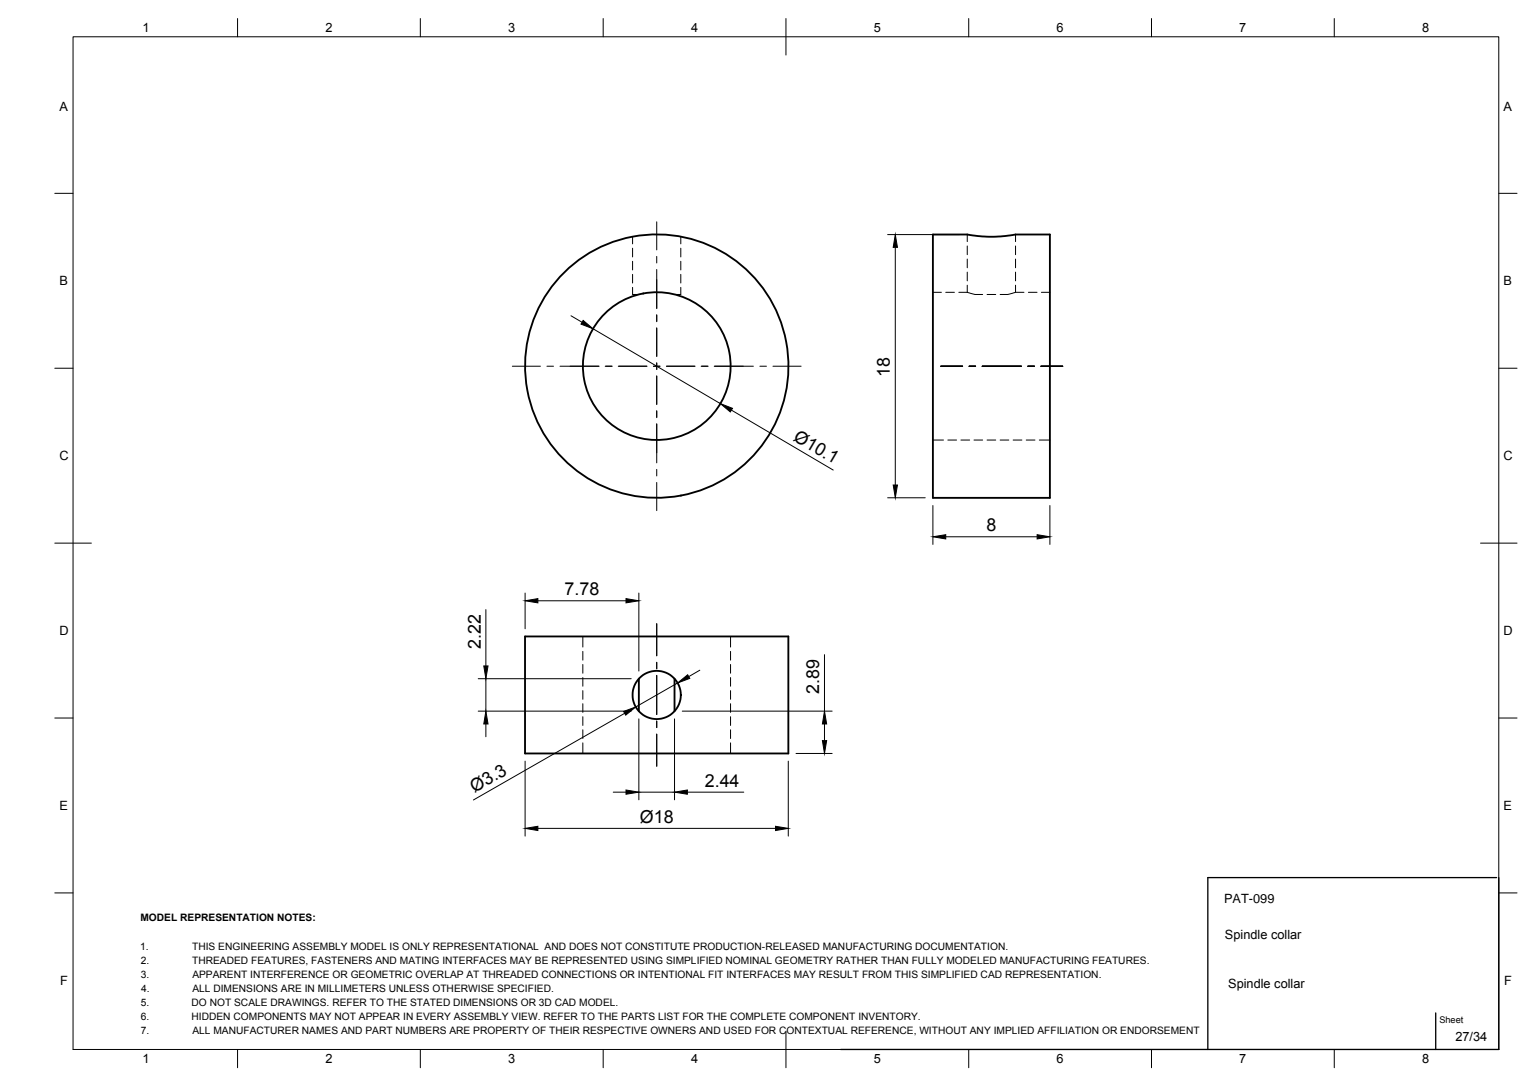
ISO-10303-21;
HEADER;
/* Generated by software containing ST-Developer
 * from STEP Tools, Inc. (www.steptools.com) 
 */

FILE_DESCRIPTION(
/* description */ ('PAT-099'),
/* implementation_level */ '2;1');

FILE_NAME(
/* name */ 'Spindle collar.step',
/* time_stamp */ '2026-10-29T17:25:42-07:00',
/* author */ (''),
/* organization */ (''),
/* preprocessor_version */ 'ST-DEVELOPER v20.2',
/* originating_system */ 'Autodesk Translation Framework v15.17.0.0',
/* authorisation */ '');

FILE_SCHEMA (('AUTOMOTIVE_DESIGN { 1 0 10303 214 3 1 1 }'));
ENDSEC;

DATA;
#10=MECHANICAL_DESIGN_GEOMETRIC_PRESENTATION_REPRESENTATION('',(#349),#11035);
#264=B_SPLINE_CURVE_WITH_KNOTS('',3,(#9974,#9975,#9976,#9977,#9978,#9979,
#9980,#9981,#9982,#9983,#9984,#9985,#9986,#9987),.UNSPECIFIED.,.F.,.F.,
(4,2,2,2,2,2,4),(0.618551524396293,0.626563103102765,0.689203386094988,
0.751843669087211,0.814483952079434,0.877124235071657,0.88513581377813),
 .UNSPECIFIED.);
#265=B_SPLINE_CURVE_WITH_KNOTS('',3,(#9991,#9992,#9993,#9994,#9995,#9996,
#9997,#9998),.UNSPECIFIED.,.F.,.F.,(4,2,2,4),(0.250614556362404,0.313254839354627,
0.37589512234685,0.383906701053323),.UNSPECIFIED.);
#266=B_SPLINE_CURVE_WITH_KNOTS('',3,(#10002,#10003,#10004,#10005,#10006,
#10007,#10008,#10009,#10010,#10011,#10012,#10013,#10014,#10015,#10016,#10017,
#10018,#10019,#10020,#10021,#10022,#10023,#10024,#10025,#10026,#10027),
 .UNSPECIFIED.,.F.,.F.,(4,2,2,2,2,2,2,2,2,2,2,2,4),(0.,0.0623062782223143,
0.124612556444629,0.186916384615149,0.249220212785669,0.31152404095619,
0.37382786912671,0.436134147349024,0.498440425571339,0.560746703793653,
0.623052982015967,0.685356810186488,0.747660638357008),.UNSPECIFIED.);
#267=B_SPLINE_CURVE_WITH_KNOTS('',3,(#10028,#10029,#10030,#10031,#10032,
#10033,#10034,#10035,#10036,#10037),.UNSPECIFIED.,.F.,.F.,(4,2,2,2,4),(0.747660638357008,
0.809964466527528,0.872268294698049,0.934574572920363,0.996880851142677),
 .UNSPECIFIED.);
#268=B_SPLINE_CURVE_WITH_KNOTS('',3,(#10038,#10039,#10040,#10041,#10042,
#10043,#10044,#10045),.UNSPECIFIED.,.F.,.F.,(4,2,2,4),(0.117322411671485,
0.125333990377958,0.187974273370181,0.250614556362404),.UNSPECIFIED.);
#299=SHAPE_REPRESENTATION_RELATIONSHIP('SRR','None',#11169,#324);
#324=ADVANCED_BREP_SHAPE_REPRESENTATION('',(#381),#11019);
#349=STYLED_ITEM('',(#11379),#381);
#381=MANIFOLD_SOLID_BREP('Body1',#4718);
#495=FACE_BOUND('',#1197,.T.);
#496=FACE_BOUND('',#1199,.T.);
#497=FACE_BOUND('',#1201,.T.);
#498=FACE_BOUND('',#1203,.T.);
#597=PLANE('',#5364);
#598=PLANE('',#5368);
#599=PLANE('',#5375);
#600=PLANE('',#5376);
#818=FACE_OUTER_BOUND('',#1193,.T.);
#819=FACE_OUTER_BOUND('',#1194,.T.);
#820=FACE_OUTER_BOUND('',#1195,.T.);
#821=FACE_OUTER_BOUND('',#1196,.T.);
#822=FACE_OUTER_BOUND('',#1198,.T.);
#823=FACE_OUTER_BOUND('',#1200,.T.);
#824=FACE_OUTER_BOUND('',#1202,.T.);
#1193=EDGE_LOOP('',(#3815,#3816));
#1194=EDGE_LOOP('',(#3817,#3818,#3819,#3820,#3821,#3822,#3823,#3824,#3825));
#1195=EDGE_LOOP('',(#3826,#3827));
#1196=EDGE_LOOP('',(#3828,#3829,#3830,#3831));
#1197=EDGE_LOOP('',(#3832,#3833,#3834,#3835,#3836));
#1198=EDGE_LOOP('',(#3837,#3838,#3839,#3840));
#1199=EDGE_LOOP('',(#3841,#3842));
#1200=EDGE_LOOP('',(#3843));
#1201=EDGE_LOOP('',(#3844));
#1202=EDGE_LOOP('',(#3845));
#1203=EDGE_LOOP('',(#3846));
#1491=LINE('',#9970,#1743);
#1492=LINE('',#10000,#1744);
#1493=LINE('',#10047,#1745);
#1494=LINE('',#10052,#1746);
#1495=LINE('',#10058,#1747);
#1743=VECTOR('',#6514,1.);
#1744=VECTOR('',#6521,0.165);
#1745=VECTOR('',#6524,1.);
#1746=VECTOR('',#6529,0.505);
#1747=VECTOR('',#6536,0.9);
#2018=CIRCLE('',#5365,0.165);
#2019=CIRCLE('',#5367,0.165);
#2020=CIRCLE('',#5370,0.505);
#2021=CIRCLE('',#5371,0.505);
#2022=CIRCLE('',#5373,0.9);
#2023=CIRCLE('',#5374,0.9);
#2369=VERTEX_POINT('',#9968);
#2370=VERTEX_POINT('',#9969);
#2371=VERTEX_POINT('',#9973);
#2372=VERTEX_POINT('',#9988);
#2373=VERTEX_POINT('',#9990);
#2374=VERTEX_POINT('',#9999);
#2375=VERTEX_POINT('',#10001);
#2376=VERTEX_POINT('',#10049);
#2377=VERTEX_POINT('',#10051);
#2378=VERTEX_POINT('',#10055);
#2379=VERTEX_POINT('',#10057);
#2884=EDGE_CURVE('',#2369,#2370,#1491,.T.);
#2885=EDGE_CURVE('',#2369,#2370,#2018,.T.);
#2886=EDGE_CURVE('',#2371,#2369,#264,.T.);
#2887=EDGE_CURVE('',#2372,#2371,#2019,.T.);
#2888=EDGE_CURVE('',#2373,#2372,#265,.T.);
#2889=EDGE_CURVE('',#2373,#2374,#1492,.T.);
#2890=EDGE_CURVE('',#2375,#2374,#266,.T.);
#2891=EDGE_CURVE('',#2374,#2375,#267,.T.);
#2892=EDGE_CURVE('',#2370,#2373,#268,.T.);
#2893=EDGE_CURVE('',#2372,#2371,#1493,.T.);
#2894=EDGE_CURVE('',#2376,#2376,#2020,.T.);
#2895=EDGE_CURVE('',#2376,#2377,#1494,.T.);
#2896=EDGE_CURVE('',#2377,#2377,#2021,.T.);
#2897=EDGE_CURVE('',#2378,#2378,#2022,.T.);
#2898=EDGE_CURVE('',#2378,#2379,#1495,.T.);
#2899=EDGE_CURVE('',#2379,#2379,#2023,.T.);
#3815=ORIENTED_EDGE('',*,*,#2884,.F.);
#3816=ORIENTED_EDGE('',*,*,#2885,.T.);
#3817=ORIENTED_EDGE('',*,*,#2886,.F.);
#3818=ORIENTED_EDGE('',*,*,#2887,.F.);
#3819=ORIENTED_EDGE('',*,*,#2888,.F.);
#3820=ORIENTED_EDGE('',*,*,#2889,.T.);
#3821=ORIENTED_EDGE('',*,*,#2890,.F.);
#3822=ORIENTED_EDGE('',*,*,#2891,.F.);
#3823=ORIENTED_EDGE('',*,*,#2889,.F.);
#3824=ORIENTED_EDGE('',*,*,#2892,.F.);
#3825=ORIENTED_EDGE('',*,*,#2885,.F.);
#3826=ORIENTED_EDGE('',*,*,#2893,.F.);
#3827=ORIENTED_EDGE('',*,*,#2887,.T.);
#3828=ORIENTED_EDGE('',*,*,#2894,.F.);
#3829=ORIENTED_EDGE('',*,*,#2895,.T.);
#3830=ORIENTED_EDGE('',*,*,#2896,.T.);
#3831=ORIENTED_EDGE('',*,*,#2895,.F.);
#3832=ORIENTED_EDGE('',*,*,#2892,.T.);
#3833=ORIENTED_EDGE('',*,*,#2888,.T.);
#3834=ORIENTED_EDGE('',*,*,#2893,.T.);
#3835=ORIENTED_EDGE('',*,*,#2886,.T.);
#3836=ORIENTED_EDGE('',*,*,#2884,.T.);
#3837=ORIENTED_EDGE('',*,*,#2897,.F.);
#3838=ORIENTED_EDGE('',*,*,#2898,.T.);
#3839=ORIENTED_EDGE('',*,*,#2899,.T.);
#3840=ORIENTED_EDGE('',*,*,#2898,.F.);
#3841=ORIENTED_EDGE('',*,*,#2890,.T.);
#3842=ORIENTED_EDGE('',*,*,#2891,.T.);
#3843=ORIENTED_EDGE('',*,*,#2897,.T.);
#3844=ORIENTED_EDGE('',*,*,#2894,.T.);
#3845=ORIENTED_EDGE('',*,*,#2899,.F.);
#3846=ORIENTED_EDGE('',*,*,#2896,.F.);
#4390=CYLINDRICAL_SURFACE('',#5366,0.165);
#4391=CYLINDRICAL_SURFACE('',#5369,0.505);
#4392=CYLINDRICAL_SURFACE('',#5372,0.9);
#4583=ADVANCED_FACE('',(#818),#597,.T.);
#4584=ADVANCED_FACE('',(#819),#4390,.F.);
#4585=ADVANCED_FACE('',(#820),#598,.T.);
#4586=ADVANCED_FACE('',(#821,#495),#4391,.F.);
#4587=ADVANCED_FACE('',(#822,#496),#4392,.T.);
#4588=ADVANCED_FACE('',(#823,#497),#599,.T.);
#4589=ADVANCED_FACE('',(#824,#498),#600,.F.);
#4718=CLOSED_SHELL('',(#4583,#4584,#4585,#4586,#4587,#4588,#4589));
#5363=AXIS2_PLACEMENT_3D('',#9966,#6510,#6511);
#5364=AXIS2_PLACEMENT_3D('',#9967,#6512,#6513);
#5365=AXIS2_PLACEMENT_3D('',#9971,#6515,#6516);
#5366=AXIS2_PLACEMENT_3D('',#9972,#6517,#6518);
#5367=AXIS2_PLACEMENT_3D('',#9989,#6519,#6520);
#5368=AXIS2_PLACEMENT_3D('',#10046,#6522,#6523);
#5369=AXIS2_PLACEMENT_3D('',#10048,#6525,#6526);
#5370=AXIS2_PLACEMENT_3D('',#10050,#6527,#6528);
#5371=AXIS2_PLACEMENT_3D('',#10053,#6530,#6531);
#5372=AXIS2_PLACEMENT_3D('',#10054,#6532,#6533);
#5373=AXIS2_PLACEMENT_3D('',#10056,#6534,#6535);
#5374=AXIS2_PLACEMENT_3D('',#10059,#6537,#6538);
#5375=AXIS2_PLACEMENT_3D('',#10060,#6539,#6540);
#5376=AXIS2_PLACEMENT_3D('',#10061,#6541,#6542);
#6510=DIRECTION('axis',(0.,0.,1.));
#6511=DIRECTION('refdir',(1.,0.,0.));
#6512=DIRECTION('center_axis',(1.,0.,0.));
#6513=DIRECTION('ref_axis',(0.,0.,-1.));
#6514=DIRECTION('',(0.,0.,1.));
#6515=DIRECTION('center_axis',(1.,0.,0.));
#6516=DIRECTION('ref_axis',(0.,0.,-1.));
#6517=DIRECTION('center_axis',(1.,0.,0.));
#6518=DIRECTION('ref_axis',(0.,0.,-1.));
#6519=DIRECTION('center_axis',(1.,0.,0.));
#6520=DIRECTION('ref_axis',(0.,0.,-1.));
#6521=DIRECTION('',(1.,0.,0.));
#6522=DIRECTION('center_axis',(1.,0.,0.));
#6523=DIRECTION('ref_axis',(0.,0.,-1.));
#6524=DIRECTION('',(0.,0.,-1.));
#6525=DIRECTION('center_axis',(0.,0.,1.));
#6526=DIRECTION('ref_axis',(1.,0.,0.));
#6527=DIRECTION('center_axis',(0.,0.,-1.));
#6528=DIRECTION('ref_axis',(1.,0.,0.));
#6529=DIRECTION('',(0.,0.,-1.));
#6530=DIRECTION('center_axis',(0.,0.,-1.));
#6531=DIRECTION('ref_axis',(1.,0.,0.));
#6532=DIRECTION('center_axis',(0.,0.,1.));
#6533=DIRECTION('ref_axis',(1.,0.,0.));
#6534=DIRECTION('center_axis',(0.,0.,1.));
#6535=DIRECTION('ref_axis',(1.,0.,0.));
#6536=DIRECTION('',(0.,0.,-1.));
#6537=DIRECTION('center_axis',(0.,0.,1.));
#6538=DIRECTION('ref_axis',(1.,0.,0.));
#6539=DIRECTION('center_axis',(0.,0.,1.));
#6540=DIRECTION('ref_axis',(1.,0.,0.));
#6541=DIRECTION('center_axis',(0.,0.,1.));
#6542=DIRECTION('ref_axis',(1.,0.,0.));
#9966=CARTESIAN_POINT('',(0.,0.,0.));
#9967=CARTESIAN_POINT('Origin',(0.49,0.,1.4));
#9968=CARTESIAN_POINT('',(0.49,0.122167917228706,1.28909463493591));
#9969=CARTESIAN_POINT('',(0.49,0.122167917228706,1.51090536506409));
#9970=CARTESIAN_POINT('',(0.49,0.122167917228706,1.));
#9971=CARTESIAN_POINT('Origin',(0.49,0.,1.4));
#9972=CARTESIAN_POINT('Origin',(0.49,0.,1.4));
#9973=CARTESIAN_POINT('',(0.49,-0.122167917228706,1.28909463493591));
#9974=CARTESIAN_POINT('Ctrl Pts',(0.49,-0.122167917228706,1.28909463493591));
#9975=CARTESIAN_POINT('Ctrl Pts',(0.490448531679987,-0.120368913626296,
1.28711294069536));
#9976=CARTESIAN_POINT('Ctrl Pts',(0.490895245371685,-0.118534896565231,
1.28518965877367));
#9977=CARTESIAN_POINT('Ctrl Pts',(0.494795015531646,-0.102111993019358,
1.2687667552278));
#9978=CARTESIAN_POINT('Ctrl Pts',(0.498442514607594,-0.0836597150224318,
1.25609154388858));
#9979=CARTESIAN_POINT('Ctrl Pts',(0.50357781976106,-0.0430495960471595,
1.23920409039234));
#9980=CARTESIAN_POINT('Ctrl Pts',(0.505,-0.020880094330741,1.235));
#9981=CARTESIAN_POINT('Ctrl Pts',(0.505,0.020880094330741,1.235));
#9982=CARTESIAN_POINT('Ctrl Pts',(0.50357781976106,0.0430495960471595,1.23920409039234));
#9983=CARTESIAN_POINT('Ctrl Pts',(0.498442514607594,0.0836597150224318,
1.25609154388858));
#9984=CARTESIAN_POINT('Ctrl Pts',(0.494795015531646,0.102111993019358,1.2687667552278));
#9985=CARTESIAN_POINT('Ctrl Pts',(0.490895245371684,0.118534896565231,1.28518965877367));
#9986=CARTESIAN_POINT('Ctrl Pts',(0.490448531679987,0.120368913626296,1.28711294069536));
#9987=CARTESIAN_POINT('Ctrl Pts',(0.49,0.122167917228706,1.28909463493591));
#9988=CARTESIAN_POINT('',(0.49,-0.122167917228706,1.51090536506409));
#9989=CARTESIAN_POINT('Origin',(0.49,0.,1.4));
#9990=CARTESIAN_POINT('',(0.505,-1.70422299968729E-17,1.565));
#9991=CARTESIAN_POINT('Ctrl Pts',(0.505,-6.93889390390723E-18,1.565));
#9992=CARTESIAN_POINT('Ctrl Pts',(0.505,-0.020880094330741,1.565));
#9993=CARTESIAN_POINT('Ctrl Pts',(0.50357781976106,-0.0430495960471595,
1.56079590960766));
#9994=CARTESIAN_POINT('Ctrl Pts',(0.498442514607594,-0.0836597150224318,
1.54390845611142));
#9995=CARTESIAN_POINT('Ctrl Pts',(0.494795015531646,-0.102111993019358,
1.5312332447722));
#9996=CARTESIAN_POINT('Ctrl Pts',(0.490895245371684,-0.118534896565231,
1.51481034122633));
#9997=CARTESIAN_POINT('Ctrl Pts',(0.490448531679987,-0.120368913626296,
1.51288705930464));
#9998=CARTESIAN_POINT('Ctrl Pts',(0.49,-0.122167917228706,1.51090536506409));
#9999=CARTESIAN_POINT('',(0.9,-2.02066721859313E-17,1.565));
#10000=CARTESIAN_POINT('',(0.49,-2.02066721859313E-17,1.565));
#10001=CARTESIAN_POINT('',(0.884745726183518,0.165,1.4));
#10002=CARTESIAN_POINT('Ctrl Pts',(0.884745726183518,0.165,1.4));
#10003=CARTESIAN_POINT('Ctrl Pts',(0.884745726183518,0.165,1.37923124059256));
#10004=CARTESIAN_POINT('Ctrl Pts',(0.885552759505264,0.160839719007584,
1.35711110492666));
#10005=CARTESIAN_POINT('Ctrl Pts',(0.888448648150043,0.143986470216691,
1.31647293736623));
#10006=CARTESIAN_POINT('Ctrl Pts',(0.890493604851638,0.131295993814186,
1.29795075602263));
#10007=CARTESIAN_POINT('Ctrl Pts',(0.89431723432394,0.102049819008125,1.26870458121656));
#10008=CARTESIAN_POINT('Ctrl Pts',(0.896347088899543,0.0835273920906824,
1.25601365401642));
#10009=CARTESIAN_POINT('Ctrl Pts',(0.899208271860583,0.0428883760934127,
1.23916007816136));
#10010=CARTESIAN_POINT('Ctrl Pts',(0.9,0.0207679427235068,1.235));
#10011=CARTESIAN_POINT('Ctrl Pts',(0.9,-0.0207679427235068,1.235));
#10012=CARTESIAN_POINT('Ctrl Pts',(0.899208271860583,-0.0428883760934127,
1.23916007816136));
#10013=CARTESIAN_POINT('Ctrl Pts',(0.896347088899543,-0.0835273920906823,
1.25601365401642));
#10014=CARTESIAN_POINT('Ctrl Pts',(0.89431723432394,-0.102049819008125,
1.26870458121656));
#10015=CARTESIAN_POINT('Ctrl Pts',(0.890493604851638,-0.131295993814186,
1.29795075602263));
#10016=CARTESIAN_POINT('Ctrl Pts',(0.888448648150043,-0.143986470216691,
1.31647293736623));
#10017=CARTESIAN_POINT('Ctrl Pts',(0.885552759505264,-0.160839719007584,
1.35711110492666));
#10018=CARTESIAN_POINT('Ctrl Pts',(0.884745726183518,-0.165,1.37923124059256));
#10019=CARTESIAN_POINT('Ctrl Pts',(0.884745726183518,-0.165,1.42076875940744));
#10020=CARTESIAN_POINT('Ctrl Pts',(0.885552759505264,-0.160839719007584,
1.44288889507334));
#10021=CARTESIAN_POINT('Ctrl Pts',(0.888448648150043,-0.14398647021669,
1.48352706263377));
#10022=CARTESIAN_POINT('Ctrl Pts',(0.890493604851638,-0.131295993814186,
1.50204924397737));
#10023=CARTESIAN_POINT('Ctrl Pts',(0.89431723432394,-0.102049819008125,
1.53129541878344));
#10024=CARTESIAN_POINT('Ctrl Pts',(0.896347088899543,-0.0835273920906824,
1.54398634598358));
#10025=CARTESIAN_POINT('Ctrl Pts',(0.899208271860583,-0.0428883760934128,
1.56083992183864));
#10026=CARTESIAN_POINT('Ctrl Pts',(0.9,-0.0207679427235068,1.565));
#10027=CARTESIAN_POINT('Ctrl Pts',(0.9,-6.93889390390723E-18,1.565));
#10028=CARTESIAN_POINT('Ctrl Pts',(0.9,-3.46944695195361E-17,1.565));
#10029=CARTESIAN_POINT('Ctrl Pts',(0.9,0.0207679427235068,1.565));
#10030=CARTESIAN_POINT('Ctrl Pts',(0.899208271860583,0.0428883760934127,
1.56083992183864));
#10031=CARTESIAN_POINT('Ctrl Pts',(0.896347088899543,0.0835273920906824,
1.54398634598358));
#10032=CARTESIAN_POINT('Ctrl Pts',(0.89431723432394,0.102049819008125,1.53129541878344));
#10033=CARTESIAN_POINT('Ctrl Pts',(0.890493604851638,0.131295993814186,
1.50204924397737));
#10034=CARTESIAN_POINT('Ctrl Pts',(0.888448648150043,0.143986470216691,
1.48352706263377));
#10035=CARTESIAN_POINT('Ctrl Pts',(0.885552759505264,0.160839719007584,
1.44288889507334));
#10036=CARTESIAN_POINT('Ctrl Pts',(0.884745726183518,0.165,1.42076875940744));
#10037=CARTESIAN_POINT('Ctrl Pts',(0.884745726183518,0.165,1.4));
#10038=CARTESIAN_POINT('Ctrl Pts',(0.49,0.122167917228706,1.51090536506409));
#10039=CARTESIAN_POINT('Ctrl Pts',(0.490448531679987,0.120368913626296,
1.51288705930464));
#10040=CARTESIAN_POINT('Ctrl Pts',(0.490895245371685,0.118534896565231,
1.51481034122633));
#10041=CARTESIAN_POINT('Ctrl Pts',(0.494795015531646,0.102111993019358,
1.5312332447722));
#10042=CARTESIAN_POINT('Ctrl Pts',(0.498442514607594,0.0836597150224318,
1.54390845611142));
#10043=CARTESIAN_POINT('Ctrl Pts',(0.50357781976106,0.0430495960471594,
1.56079590960766));
#10044=CARTESIAN_POINT('Ctrl Pts',(0.505,0.020880094330741,1.565));
#10045=CARTESIAN_POINT('Ctrl Pts',(0.505,0.,1.565));
#10046=CARTESIAN_POINT('Origin',(0.49,0.,1.4));
#10047=CARTESIAN_POINT('',(0.49,-0.122167917228706,1.));
#10048=CARTESIAN_POINT('Origin',(0.,0.,1.));
#10049=CARTESIAN_POINT('',(-0.505,-6.18446633569413E-17,1.8));
#10050=CARTESIAN_POINT('Origin',(0.,0.,1.8));
#10051=CARTESIAN_POINT('',(-0.505,-6.18446633569413E-17,1.));
#10052=CARTESIAN_POINT('',(-0.505,-6.18446633569413E-17,1.));
#10053=CARTESIAN_POINT('Origin',(0.,0.,1.));
#10054=CARTESIAN_POINT('Origin',(0.,0.,1.));
#10055=CARTESIAN_POINT('',(-0.9,-1.10218211923262E-16,1.8));
#10056=CARTESIAN_POINT('Origin',(0.,0.,1.8));
#10057=CARTESIAN_POINT('',(-0.9,-1.10218211923262E-16,1.));
#10058=CARTESIAN_POINT('',(-0.9,-1.10218211923262E-16,1.));
#10059=CARTESIAN_POINT('Origin',(0.,0.,1.));
#10060=CARTESIAN_POINT('Origin',(0.,0.,1.8));
#10061=CARTESIAN_POINT('Origin',(0.,0.,1.));
#10986=UNCERTAINTY_MEASURE_WITH_UNIT(LENGTH_MEASURE(0.001),#11036,
'DISTANCE_ACCURACY_VALUE',
'Maximum model space distance between geometric entities at asserted c
onnectivities');
#11002=UNCERTAINTY_MEASURE_WITH_UNIT(LENGTH_MEASURE(0.001),#11036,
'DISTANCE_ACCURACY_VALUE',
'Maximum model space distance between geometric entities at asserted c
onnectivities');
#11019=(
GEOMETRIC_REPRESENTATION_CONTEXT(3)
GLOBAL_UNCERTAINTY_ASSIGNED_CONTEXT((#10986))
GLOBAL_UNIT_ASSIGNED_CONTEXT((#11036,#11038,#11039))
REPRESENTATION_CONTEXT('','3D')
);
#11035=(
GEOMETRIC_REPRESENTATION_CONTEXT(3)
GLOBAL_UNCERTAINTY_ASSIGNED_CONTEXT((#11002))
GLOBAL_UNIT_ASSIGNED_CONTEXT((#11036,#11038,#11039))
REPRESENTATION_CONTEXT('','3D')
);
#11036=(
LENGTH_UNIT()
NAMED_UNIT(*)
SI_UNIT(.CENTI.,.METRE.)
);
#11038=(
NAMED_UNIT(*)
PLANE_ANGLE_UNIT()
SI_UNIT($,.RADIAN.)
);
#11039=(
NAMED_UNIT(*)
SI_UNIT($,.STERADIAN.)
SOLID_ANGLE_UNIT()
);
#11056=SHAPE_DEFINITION_REPRESENTATION(#11090,#11169);
#11090=PRODUCT_DEFINITION_SHAPE('',$,#11202);
#11169=SHAPE_REPRESENTATION('',(#5363),#11019);
#11185=PRODUCT_DEFINITION_CONTEXT('part definition',#11283,'design');
#11202=PRODUCT_DEFINITION('Spindle collar','Spindle collar',#11234,#11185);
#11234=PRODUCT_DEFINITION_FORMATION('',$,#11301);
#11283=APPLICATION_CONTEXT(
'Core Data for Automotive Mechanical Design Process');
#11284=PRODUCT_CONTEXT('part definition',#11283,'mechanical');
#11301=PRODUCT('Spindle collar','Spindle collar','Spindle collar',(#11284));
#11373=COLOUR_RGB('Sky Blue',0.24,0.69,0.87);
#11374=FILL_AREA_STYLE_COLOUR('',#11373);
#11375=FILL_AREA_STYLE('',(#11374));
#11376=SURFACE_STYLE_FILL_AREA(#11375);
#11377=SURFACE_SIDE_STYLE('',(#11376));
#11378=SURFACE_STYLE_USAGE(.BOTH.,#11377);
#11379=PRESENTATION_STYLE_ASSIGNMENT((#11378));
ENDSEC;
END-ISO-10303-21;
